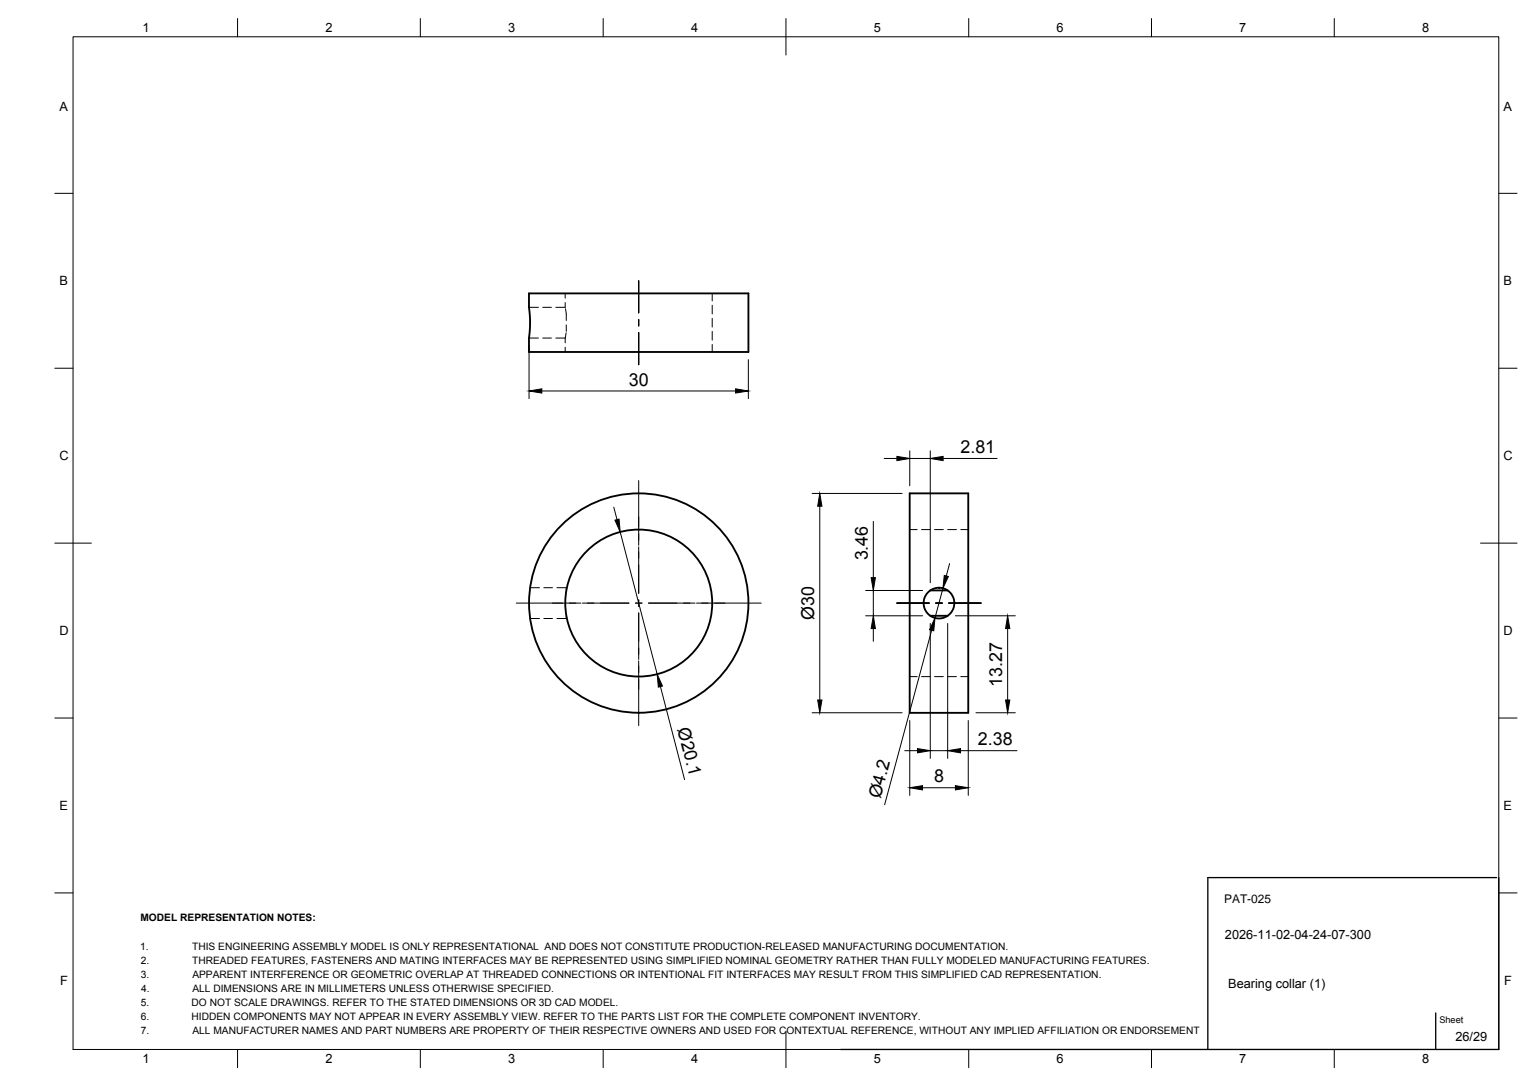
ISO-10303-21;
HEADER;
/* Generated by software containing ST-Developer
 * from STEP Tools, Inc. (www.steptools.com) 
 */

FILE_DESCRIPTION(
/* description */ ('Counter shaft with two pulleys and keyed hub'),
/* implementation_level */ '2;1');

FILE_NAME(
/* name */ 'Bearing collar (1).step',
/* time_stamp */ '2026-10-27T10:46:10-07:00',
/* author */ (''),
/* organization */ (''),
/* preprocessor_version */ 'ST-DEVELOPER v20.2',
/* originating_system */ 'Autodesk Translation Framework v15.17.0.0',
/* authorisation */ '');

FILE_SCHEMA (('AUTOMOTIVE_DESIGN { 1 0 10303 214 3 1 1 }'));
ENDSEC;

DATA;
#10=MECHANICAL_DESIGN_GEOMETRIC_PRESENTATION_REPRESENTATION('',(#310),#10821);
#216=B_SPLINE_CURVE_WITH_KNOTS('',3,(#9611,#9612,#9613,#9614,#9615,#9616,
#9617,#9618,#9619,#9620,#9621,#9622,#9623,#9624),.UNSPECIFIED.,.F.,.F.,
(4,2,2,2,2,2,4),(0.756005737987019,0.793568827564645,0.8729225200542,0.952276212543755,
1.03162990503331,1.11098359752287,1.14854668710049),.UNSPECIFIED.);
#217=B_SPLINE_CURVE_WITH_KNOTS('',3,(#9630,#9631,#9632,#9633,#9634,#9635,
#9636,#9637,#9638,#9639,#9640,#9641,#9642,#9643,#9644,#9645,#9646,#9647),
 .UNSPECIFIED.,.F.,.F.,(4,2,2,2,2,2,2,2,4),(0.,0.0792165807733624,0.158433161546725,
0.237648697074569,0.316864232602414,0.396079768130259,0.475295303658103,
0.554511884431466,0.633728465204828),.UNSPECIFIED.);
#218=B_SPLINE_CURVE_WITH_KNOTS('',3,(#9648,#9649,#9650,#9651,#9652,#9653,
#9654,#9655,#9656,#9657,#9658,#9659,#9660,#9661,#9662,#9663,#9664,#9665),
 .UNSPECIFIED.,.F.,.F.,(4,2,2,2,2,2,2,2,4),(0.633728465204828,0.712945045978191,
0.792161626751553,0.871377162279398,0.950592697807242,1.02980823333509,
1.10902376886293,1.18824034963629,1.26745693040966),.UNSPECIFIED.);
#219=B_SPLINE_CURVE_WITH_KNOTS('',3,(#9668,#9669,#9670,#9671,#9672,#9673,
#9674,#9675,#9676,#9677,#9678,#9679,#9680,#9681),.UNSPECIFIED.,.F.,.F.,
(4,2,2,2,2,2,4),(0.121154929624521,0.158718019202141,0.238071711691696,
0.317425404181252,0.396779096670807,0.476132789160362,0.513695878737985),
 .UNSPECIFIED.);
#259=SHAPE_REPRESENTATION_RELATIONSHIP('SRR','None',#10947,#284);
#284=ADVANCED_BREP_SHAPE_REPRESENTATION('',(#335),#10815);
#310=STYLED_ITEM('',(#11135),#335);
#335=MANIFOLD_SOLID_BREP('Body1',#5594);
#413=FACE_BOUND('',#1141,.T.);
#414=FACE_BOUND('',#1143,.T.);
#415=FACE_BOUND('',#1145,.T.);
#416=FACE_BOUND('',#1147,.T.);
#536=PLANE('',#6193);
#537=PLANE('',#6198);
#538=PLANE('',#6205);
#539=PLANE('',#6206);
#750=FACE_OUTER_BOUND('',#1137,.T.);
#751=FACE_OUTER_BOUND('',#1138,.T.);
#752=FACE_OUTER_BOUND('',#1139,.T.);
#753=FACE_OUTER_BOUND('',#1140,.T.);
#754=FACE_OUTER_BOUND('',#1142,.T.);
#755=FACE_OUTER_BOUND('',#1144,.T.);
#756=FACE_OUTER_BOUND('',#1146,.T.);
#1137=EDGE_LOOP('',(#4301,#4302));
#1138=EDGE_LOOP('',(#4303,#4304,#4305,#4306,#4307,#4308,#4309,#4310,#4311));
#1139=EDGE_LOOP('',(#4312,#4313,#4314));
#1140=EDGE_LOOP('',(#4315,#4316,#4317,#4318));
#1141=EDGE_LOOP('',(#4319,#4320,#4321,#4322));
#1142=EDGE_LOOP('',(#4323,#4324,#4325,#4326));
#1143=EDGE_LOOP('',(#4327,#4328));
#1144=EDGE_LOOP('',(#4329));
#1145=EDGE_LOOP('',(#4330));
#1146=EDGE_LOOP('',(#4331));
#1147=EDGE_LOOP('',(#4332));
#1500=LINE('',#9607,#1889);
#1501=LINE('',#9628,#1890);
#1502=LINE('',#9683,#1891);
#1503=LINE('',#9688,#1892);
#1504=LINE('',#9694,#1893);
#1889=VECTOR('',#7386,1.);
#1890=VECTOR('',#7393,0.21);
#1891=VECTOR('',#7398,1.);
#1892=VECTOR('',#7403,1.005);
#1893=VECTOR('',#7410,1.5);
#2196=CIRCLE('',#6194,0.21);
#2197=CIRCLE('',#6196,0.21);
#2198=CIRCLE('',#6197,0.21);
#2199=CIRCLE('',#6200,1.005);
#2200=CIRCLE('',#6201,1.005);
#2201=CIRCLE('',#6203,1.5);
#2202=CIRCLE('',#6204,1.5);
#2615=VERTEX_POINT('',#9605);
#2616=VERTEX_POINT('',#9606);
#2617=VERTEX_POINT('',#9610);
#2618=VERTEX_POINT('',#9625);
#2619=VERTEX_POINT('',#9627);
#2620=VERTEX_POINT('',#9629);
#2621=VERTEX_POINT('',#9666);
#2622=VERTEX_POINT('',#9685);
#2623=VERTEX_POINT('',#9687);
#2624=VERTEX_POINT('',#9691);
#2625=VERTEX_POINT('',#9693);
#3223=EDGE_CURVE('',#2615,#2616,#1500,.T.);
#3224=EDGE_CURVE('',#2615,#2616,#2196,.T.);
#3225=EDGE_CURVE('',#2617,#2615,#216,.T.);
#3226=EDGE_CURVE('',#2618,#2617,#2197,.T.);
#3227=EDGE_CURVE('',#2618,#2619,#1501,.T.);
#3228=EDGE_CURVE('',#2620,#2619,#217,.T.);
#3229=EDGE_CURVE('',#2619,#2620,#218,.T.);
#3230=EDGE_CURVE('',#2621,#2618,#2198,.T.);
#3231=EDGE_CURVE('',#2616,#2621,#219,.T.);
#3232=EDGE_CURVE('',#2621,#2617,#1502,.T.);
#3233=EDGE_CURVE('',#2622,#2622,#2199,.T.);
#3234=EDGE_CURVE('',#2622,#2623,#1503,.T.);
#3235=EDGE_CURVE('',#2623,#2623,#2200,.T.);
#3236=EDGE_CURVE('',#2624,#2624,#2201,.T.);
#3237=EDGE_CURVE('',#2624,#2625,#1504,.T.);
#3238=EDGE_CURVE('',#2625,#2625,#2202,.T.);
#4301=ORIENTED_EDGE('',*,*,#3223,.F.);
#4302=ORIENTED_EDGE('',*,*,#3224,.T.);
#4303=ORIENTED_EDGE('',*,*,#3225,.F.);
#4304=ORIENTED_EDGE('',*,*,#3226,.F.);
#4305=ORIENTED_EDGE('',*,*,#3227,.T.);
#4306=ORIENTED_EDGE('',*,*,#3228,.F.);
#4307=ORIENTED_EDGE('',*,*,#3229,.F.);
#4308=ORIENTED_EDGE('',*,*,#3227,.F.);
#4309=ORIENTED_EDGE('',*,*,#3230,.F.);
#4310=ORIENTED_EDGE('',*,*,#3231,.F.);
#4311=ORIENTED_EDGE('',*,*,#3224,.F.);
#4312=ORIENTED_EDGE('',*,*,#3232,.F.);
#4313=ORIENTED_EDGE('',*,*,#3230,.T.);
#4314=ORIENTED_EDGE('',*,*,#3226,.T.);
#4315=ORIENTED_EDGE('',*,*,#3233,.F.);
#4316=ORIENTED_EDGE('',*,*,#3234,.T.);
#4317=ORIENTED_EDGE('',*,*,#3235,.T.);
#4318=ORIENTED_EDGE('',*,*,#3234,.F.);
#4319=ORIENTED_EDGE('',*,*,#3231,.T.);
#4320=ORIENTED_EDGE('',*,*,#3232,.T.);
#4321=ORIENTED_EDGE('',*,*,#3225,.T.);
#4322=ORIENTED_EDGE('',*,*,#3223,.T.);
#4323=ORIENTED_EDGE('',*,*,#3236,.F.);
#4324=ORIENTED_EDGE('',*,*,#3237,.T.);
#4325=ORIENTED_EDGE('',*,*,#3238,.T.);
#4326=ORIENTED_EDGE('',*,*,#3237,.F.);
#4327=ORIENTED_EDGE('',*,*,#3228,.T.);
#4328=ORIENTED_EDGE('',*,*,#3229,.T.);
#4329=ORIENTED_EDGE('',*,*,#3236,.T.);
#4330=ORIENTED_EDGE('',*,*,#3233,.T.);
#4331=ORIENTED_EDGE('',*,*,#3238,.F.);
#4332=ORIENTED_EDGE('',*,*,#3235,.F.);
#5165=CYLINDRICAL_SURFACE('',#6195,0.21);
#5166=CYLINDRICAL_SURFACE('',#6199,1.005);
#5167=CYLINDRICAL_SURFACE('',#6202,1.5);
#5421=ADVANCED_FACE('',(#750),#536,.T.);
#5422=ADVANCED_FACE('',(#751),#5165,.F.);
#5423=ADVANCED_FACE('',(#752),#537,.T.);
#5424=ADVANCED_FACE('',(#753,#413),#5166,.F.);
#5425=ADVANCED_FACE('',(#754,#414),#5167,.T.);
#5426=ADVANCED_FACE('',(#755,#415),#538,.T.);
#5427=ADVANCED_FACE('',(#756,#416),#539,.F.);
#5594=CLOSED_SHELL('',(#5421,#5422,#5423,#5424,#5425,#5426,#5427));
#6192=AXIS2_PLACEMENT_3D('',#9603,#7382,#7383);
#6193=AXIS2_PLACEMENT_3D('',#9604,#7384,#7385);
#6194=AXIS2_PLACEMENT_3D('',#9608,#7387,#7388);
#6195=AXIS2_PLACEMENT_3D('',#9609,#7389,#7390);
#6196=AXIS2_PLACEMENT_3D('',#9626,#7391,#7392);
#6197=AXIS2_PLACEMENT_3D('',#9667,#7394,#7395);
#6198=AXIS2_PLACEMENT_3D('',#9682,#7396,#7397);
#6199=AXIS2_PLACEMENT_3D('',#9684,#7399,#7400);
#6200=AXIS2_PLACEMENT_3D('',#9686,#7401,#7402);
#6201=AXIS2_PLACEMENT_3D('',#9689,#7404,#7405);
#6202=AXIS2_PLACEMENT_3D('',#9690,#7406,#7407);
#6203=AXIS2_PLACEMENT_3D('',#9692,#7408,#7409);
#6204=AXIS2_PLACEMENT_3D('',#9695,#7411,#7412);
#6205=AXIS2_PLACEMENT_3D('',#9696,#7413,#7414);
#6206=AXIS2_PLACEMENT_3D('',#9697,#7415,#7416);
#7382=DIRECTION('axis',(0.,0.,1.));
#7383=DIRECTION('refdir',(1.,0.,0.));
#7384=DIRECTION('center_axis',(0.,0.,1.));
#7385=DIRECTION('ref_axis',(1.,0.,0.));
#7386=DIRECTION('',(0.,1.,0.));
#7387=DIRECTION('center_axis',(0.,0.,1.));
#7388=DIRECTION('ref_axis',(1.,0.,0.));
#7389=DIRECTION('center_axis',(0.,0.,1.));
#7390=DIRECTION('ref_axis',(1.,0.,0.));
#7391=DIRECTION('center_axis',(0.,0.,1.));
#7392=DIRECTION('ref_axis',(1.,0.,0.));
#7393=DIRECTION('',(0.,0.,1.));
#7394=DIRECTION('center_axis',(0.,0.,1.));
#7395=DIRECTION('ref_axis',(1.,0.,0.));
#7396=DIRECTION('center_axis',(0.,0.,1.));
#7397=DIRECTION('ref_axis',(1.,0.,0.));
#7398=DIRECTION('',(0.,-1.,0.));
#7399=DIRECTION('center_axis',(0.,1.,0.));
#7400=DIRECTION('ref_axis',(1.,0.,0.));
#7401=DIRECTION('center_axis',(0.,-1.,0.));
#7402=DIRECTION('ref_axis',(1.,0.,0.));
#7403=DIRECTION('',(0.,-1.,0.));
#7404=DIRECTION('center_axis',(0.,-1.,0.));
#7405=DIRECTION('ref_axis',(1.,0.,0.));
#7406=DIRECTION('center_axis',(0.,1.,0.));
#7407=DIRECTION('ref_axis',(1.,0.,0.));
#7408=DIRECTION('center_axis',(0.,1.,0.));
#7409=DIRECTION('ref_axis',(1.,0.,0.));
#7410=DIRECTION('',(0.,-1.,0.));
#7411=DIRECTION('center_axis',(0.,1.,0.));
#7412=DIRECTION('ref_axis',(1.,0.,0.));
#7413=DIRECTION('center_axis',(0.,1.,0.));
#7414=DIRECTION('ref_axis',(1.,0.,0.));
#7415=DIRECTION('center_axis',(0.,1.,0.));
#7416=DIRECTION('ref_axis',(1.,0.,0.));
#9603=CARTESIAN_POINT('',(0.,0.,0.));
#9604=CARTESIAN_POINT('Origin',(0.,22.85,5.52));
#9605=CARTESIAN_POINT('',(0.172988438920056,22.7309411910021,5.52));
#9606=CARTESIAN_POINT('',(0.172988438920056,22.9690588089979,5.52));
#9607=CARTESIAN_POINT('',(0.172988438920056,22.45,5.52));
#9608=CARTESIAN_POINT('Origin',(0.,22.85,5.52));
#9609=CARTESIAN_POINT('Origin',(0.,22.85,5.52));
#9610=CARTESIAN_POINT('',(-0.172988438920056,22.7309411910021,5.52));
#9611=CARTESIAN_POINT('Ctrl Pts',(-0.172988438920058,22.7309411910021,5.52));
#9612=CARTESIAN_POINT('Ctrl Pts',(-0.165594865311317,22.7201985776047,5.52129192197638));
#9613=CARTESIAN_POINT('Ctrl Pts',(-0.157297138725606,22.7103122906273,5.52265394943905));
#9614=CARTESIAN_POINT('Ctrl Pts',(-0.129892073845076,22.6829072257467,5.5267480843909));
#9615=CARTESIAN_POINT('Ctrl Pts',(-0.106330167759284,22.6667579436671,5.52969589327638));
#9616=CARTESIAN_POINT('Ctrl Pts',(-0.0546129046324105,22.6453022060351,
5.53385029472357));
#9617=CARTESIAN_POINT('Ctrl Pts',(-0.0264512308298518,22.64,5.535));
#9618=CARTESIAN_POINT('Ctrl Pts',(0.0264512308298517,22.64,5.535));
#9619=CARTESIAN_POINT('Ctrl Pts',(0.0546129046324104,22.6453022060351,5.53385029472357));
#9620=CARTESIAN_POINT('Ctrl Pts',(0.106330167759284,22.6667579436671,5.52969589327638));
#9621=CARTESIAN_POINT('Ctrl Pts',(0.129892073845076,22.6829072257467,5.5267480843909));
#9622=CARTESIAN_POINT('Ctrl Pts',(0.157297138725606,22.7103122906273,5.52265394943905));
#9623=CARTESIAN_POINT('Ctrl Pts',(0.165594865311316,22.7201985776047,5.52129192197638));
#9624=CARTESIAN_POINT('Ctrl Pts',(0.172988438920056,22.7309411910021,5.52));
#9625=CARTESIAN_POINT('',(-0.21,22.85,5.52));
#9626=CARTESIAN_POINT('Origin',(0.,22.85,5.52));
#9627=CARTESIAN_POINT('',(-0.21,22.85,6.01522725533839));
#9628=CARTESIAN_POINT('',(-0.21,22.85,5.52));
#9629=CARTESIAN_POINT('',(0.21,22.85,6.01522725533839));
#9630=CARTESIAN_POINT('Ctrl Pts',(0.21,22.85,6.01522725533839));
#9631=CARTESIAN_POINT('Ctrl Pts',(0.21,22.8235944730755,6.01522725533839));
#9632=CARTESIAN_POINT('Ctrl Pts',(0.204715737269595,22.7954529259093,6.01600415954412));
#9633=CARTESIAN_POINT('Ctrl Pts',(0.18327376303633,22.7437237310949,6.01880073282317));
#9634=CARTESIAN_POINT('Ctrl Pts',(0.167117923970393,22.720133075872,6.02077897157582));
#9635=CARTESIAN_POINT('Ctrl Pts',(0.129867169887369,22.682882321789,6.02448481141327));
#9636=CARTESIAN_POINT('Ctrl Pts',(0.106276408305767,22.6667262899986,6.02645455657129));
#9637=CARTESIAN_POINT('Ctrl Pts',(0.054546851405902,22.6452841751738,6.02923165515645));
#9638=CARTESIAN_POINT('Ctrl Pts',(0.0264051785092816,22.64,6.03));
#9639=CARTESIAN_POINT('Ctrl Pts',(-0.0264051785092815,22.64,6.03));
#9640=CARTESIAN_POINT('Ctrl Pts',(-0.0545468514059018,22.6452841751738,
6.02923165515645));
#9641=CARTESIAN_POINT('Ctrl Pts',(-0.106276408305767,22.6667262899986,6.02645455657129));
#9642=CARTESIAN_POINT('Ctrl Pts',(-0.129867169887368,22.682882321789,6.02448481141327));
#9643=CARTESIAN_POINT('Ctrl Pts',(-0.167117923970393,22.720133075872,6.02077897157582));
#9644=CARTESIAN_POINT('Ctrl Pts',(-0.183273763036334,22.7437237310949,6.01880073282317));
#9645=CARTESIAN_POINT('Ctrl Pts',(-0.204715737269596,22.7954529259093,6.01600415954412));
#9646=CARTESIAN_POINT('Ctrl Pts',(-0.21,22.8235944730755,6.01522725533839));
#9647=CARTESIAN_POINT('Ctrl Pts',(-0.21,22.85,6.01522725533839));
#9648=CARTESIAN_POINT('Ctrl Pts',(-0.21,22.85,6.01522725533839));
#9649=CARTESIAN_POINT('Ctrl Pts',(-0.21,22.8764055269245,6.01522725533839));
#9650=CARTESIAN_POINT('Ctrl Pts',(-0.204715737269595,22.9045470740907,6.01600415954412));
#9651=CARTESIAN_POINT('Ctrl Pts',(-0.18327376303633,22.9562762689051,6.01880073282317));
#9652=CARTESIAN_POINT('Ctrl Pts',(-0.167117923970393,22.979866924128,6.02077897157582));
#9653=CARTESIAN_POINT('Ctrl Pts',(-0.129867169887369,23.017117678211,6.02448481141327));
#9654=CARTESIAN_POINT('Ctrl Pts',(-0.106276408305767,23.0332737100014,6.02645455657129));
#9655=CARTESIAN_POINT('Ctrl Pts',(-0.054546851405902,23.0547158248262,6.02923165515645));
#9656=CARTESIAN_POINT('Ctrl Pts',(-0.0264051785092816,23.06,6.03));
#9657=CARTESIAN_POINT('Ctrl Pts',(0.0264051785092815,23.06,6.03));
#9658=CARTESIAN_POINT('Ctrl Pts',(0.0545468514059019,23.0547158248262,6.02923165515645));
#9659=CARTESIAN_POINT('Ctrl Pts',(0.106276408305767,23.0332737100014,6.02645455657129));
#9660=CARTESIAN_POINT('Ctrl Pts',(0.129867169887368,23.017117678211,6.02448481141327));
#9661=CARTESIAN_POINT('Ctrl Pts',(0.167117923970393,22.979866924128,6.02077897157582));
#9662=CARTESIAN_POINT('Ctrl Pts',(0.18327376303633,22.9562762689051,6.01880073282317));
#9663=CARTESIAN_POINT('Ctrl Pts',(0.204715737269595,22.9045470740907,6.01600415954412));
#9664=CARTESIAN_POINT('Ctrl Pts',(0.21,22.8764055269245,6.01522725533839));
#9665=CARTESIAN_POINT('Ctrl Pts',(0.21,22.85,6.01522725533839));
#9666=CARTESIAN_POINT('',(-0.172988438920056,22.9690588089979,5.52));
#9667=CARTESIAN_POINT('Origin',(0.,22.85,5.52));
#9668=CARTESIAN_POINT('Ctrl Pts',(0.172988438920055,22.9690588089979,5.52));
#9669=CARTESIAN_POINT('Ctrl Pts',(0.165594865311314,22.9798014223953,5.52129192197638));
#9670=CARTESIAN_POINT('Ctrl Pts',(0.157297138725605,22.9896877093727,5.52265394943905));
#9671=CARTESIAN_POINT('Ctrl Pts',(0.129892073845076,23.0170927742533,5.5267480843909));
#9672=CARTESIAN_POINT('Ctrl Pts',(0.106330167759284,23.033242056333,5.52969589327638));
#9673=CARTESIAN_POINT('Ctrl Pts',(0.0546129046324105,23.0546977939649,5.53385029472357));
#9674=CARTESIAN_POINT('Ctrl Pts',(0.0264512308298518,23.06,5.535));
#9675=CARTESIAN_POINT('Ctrl Pts',(-0.0264512308298517,23.06,5.535));
#9676=CARTESIAN_POINT('Ctrl Pts',(-0.0546129046324079,23.0546977939649,
5.53385029472357));
#9677=CARTESIAN_POINT('Ctrl Pts',(-0.106330167759282,23.033242056333,5.52969589327638));
#9678=CARTESIAN_POINT('Ctrl Pts',(-0.129892073845076,23.0170927742533,5.5267480843909));
#9679=CARTESIAN_POINT('Ctrl Pts',(-0.157297138725605,22.9896877093727,5.52265394943905));
#9680=CARTESIAN_POINT('Ctrl Pts',(-0.165594865311314,22.9798014223953,5.52129192197638));
#9681=CARTESIAN_POINT('Ctrl Pts',(-0.172988438920055,22.9690588089979,5.52));
#9682=CARTESIAN_POINT('Origin',(0.,22.85,5.52));
#9683=CARTESIAN_POINT('',(-0.172988438920056,22.45,5.52));
#9684=CARTESIAN_POINT('Origin',(0.,22.45,4.53));
#9685=CARTESIAN_POINT('',(-1.005,23.25,4.53));
#9686=CARTESIAN_POINT('Origin',(0.,23.25,4.53));
#9687=CARTESIAN_POINT('',(-1.005,22.45,4.53));
#9688=CARTESIAN_POINT('',(-1.005,22.45,4.53));
#9689=CARTESIAN_POINT('Origin',(0.,22.45,4.53));
#9690=CARTESIAN_POINT('Origin',(0.,22.45,4.53));
#9691=CARTESIAN_POINT('',(-1.5,23.25,4.53));
#9692=CARTESIAN_POINT('Origin',(0.,23.25,4.53));
#9693=CARTESIAN_POINT('',(-1.5,22.45,4.53));
#9694=CARTESIAN_POINT('',(-1.5,22.45,4.53));
#9695=CARTESIAN_POINT('Origin',(0.,22.45,4.53));
#9696=CARTESIAN_POINT('Origin',(0.,23.25,4.53));
#9697=CARTESIAN_POINT('Origin',(0.,22.45,4.53));
#10785=UNCERTAINTY_MEASURE_WITH_UNIT(LENGTH_MEASURE(0.001),#10822,
'DISTANCE_ACCURACY_VALUE',
'Maximum model space distance between geometric entities at asserted c
onnectivities');
#10791=UNCERTAINTY_MEASURE_WITH_UNIT(LENGTH_MEASURE(0.001),#10822,
'DISTANCE_ACCURACY_VALUE',
'Maximum model space distance between geometric entities at asserted c
onnectivities');
#10815=(
GEOMETRIC_REPRESENTATION_CONTEXT(3)
GLOBAL_UNCERTAINTY_ASSIGNED_CONTEXT((#10785))
GLOBAL_UNIT_ASSIGNED_CONTEXT((#10822,#10824,#10825))
REPRESENTATION_CONTEXT('','3D')
);
#10821=(
GEOMETRIC_REPRESENTATION_CONTEXT(3)
GLOBAL_UNCERTAINTY_ASSIGNED_CONTEXT((#10791))
GLOBAL_UNIT_ASSIGNED_CONTEXT((#10822,#10824,#10825))
REPRESENTATION_CONTEXT('','3D')
);
#10822=(
LENGTH_UNIT()
NAMED_UNIT(*)
SI_UNIT(.CENTI.,.METRE.)
);
#10824=(
NAMED_UNIT(*)
PLANE_ANGLE_UNIT()
SI_UNIT($,.RADIAN.)
);
#10825=(
NAMED_UNIT(*)
SI_UNIT($,.STERADIAN.)
SOLID_ANGLE_UNIT()
);
#10849=SHAPE_DEFINITION_REPRESENTATION(#10897,#10947);
#10897=PRODUCT_DEFINITION_SHAPE('',$,#10977);
#10947=SHAPE_REPRESENTATION('',(#6192),#10815);
#10953=PRODUCT_DEFINITION_CONTEXT('part definition',#11042,'design');
#10977=PRODUCT_DEFINITION('Bearing collar (1)','Bearing collar (1)',#11006,
#10953);
#11006=PRODUCT_DEFINITION_FORMATION('',$,#11067);
#11042=APPLICATION_CONTEXT(
'Core Data for Automotive Mechanical Design Process');
#11043=PRODUCT_CONTEXT('part definition',#11042,'mechanical');
#11067=PRODUCT('Bearing collar (1)','Bearing collar (1)','Bearing collar (1)',
(#11043));
#11129=COLOUR_RGB('Grey',0.48,0.52,0.57);
#11130=FILL_AREA_STYLE_COLOUR('',#11129);
#11131=FILL_AREA_STYLE('',(#11130));
#11132=SURFACE_STYLE_FILL_AREA(#11131);
#11133=SURFACE_SIDE_STYLE('',(#11132));
#11134=SURFACE_STYLE_USAGE(.BOTH.,#11133);
#11135=PRESENTATION_STYLE_ASSIGNMENT((#11134));
ENDSEC;
END-ISO-10303-21;
